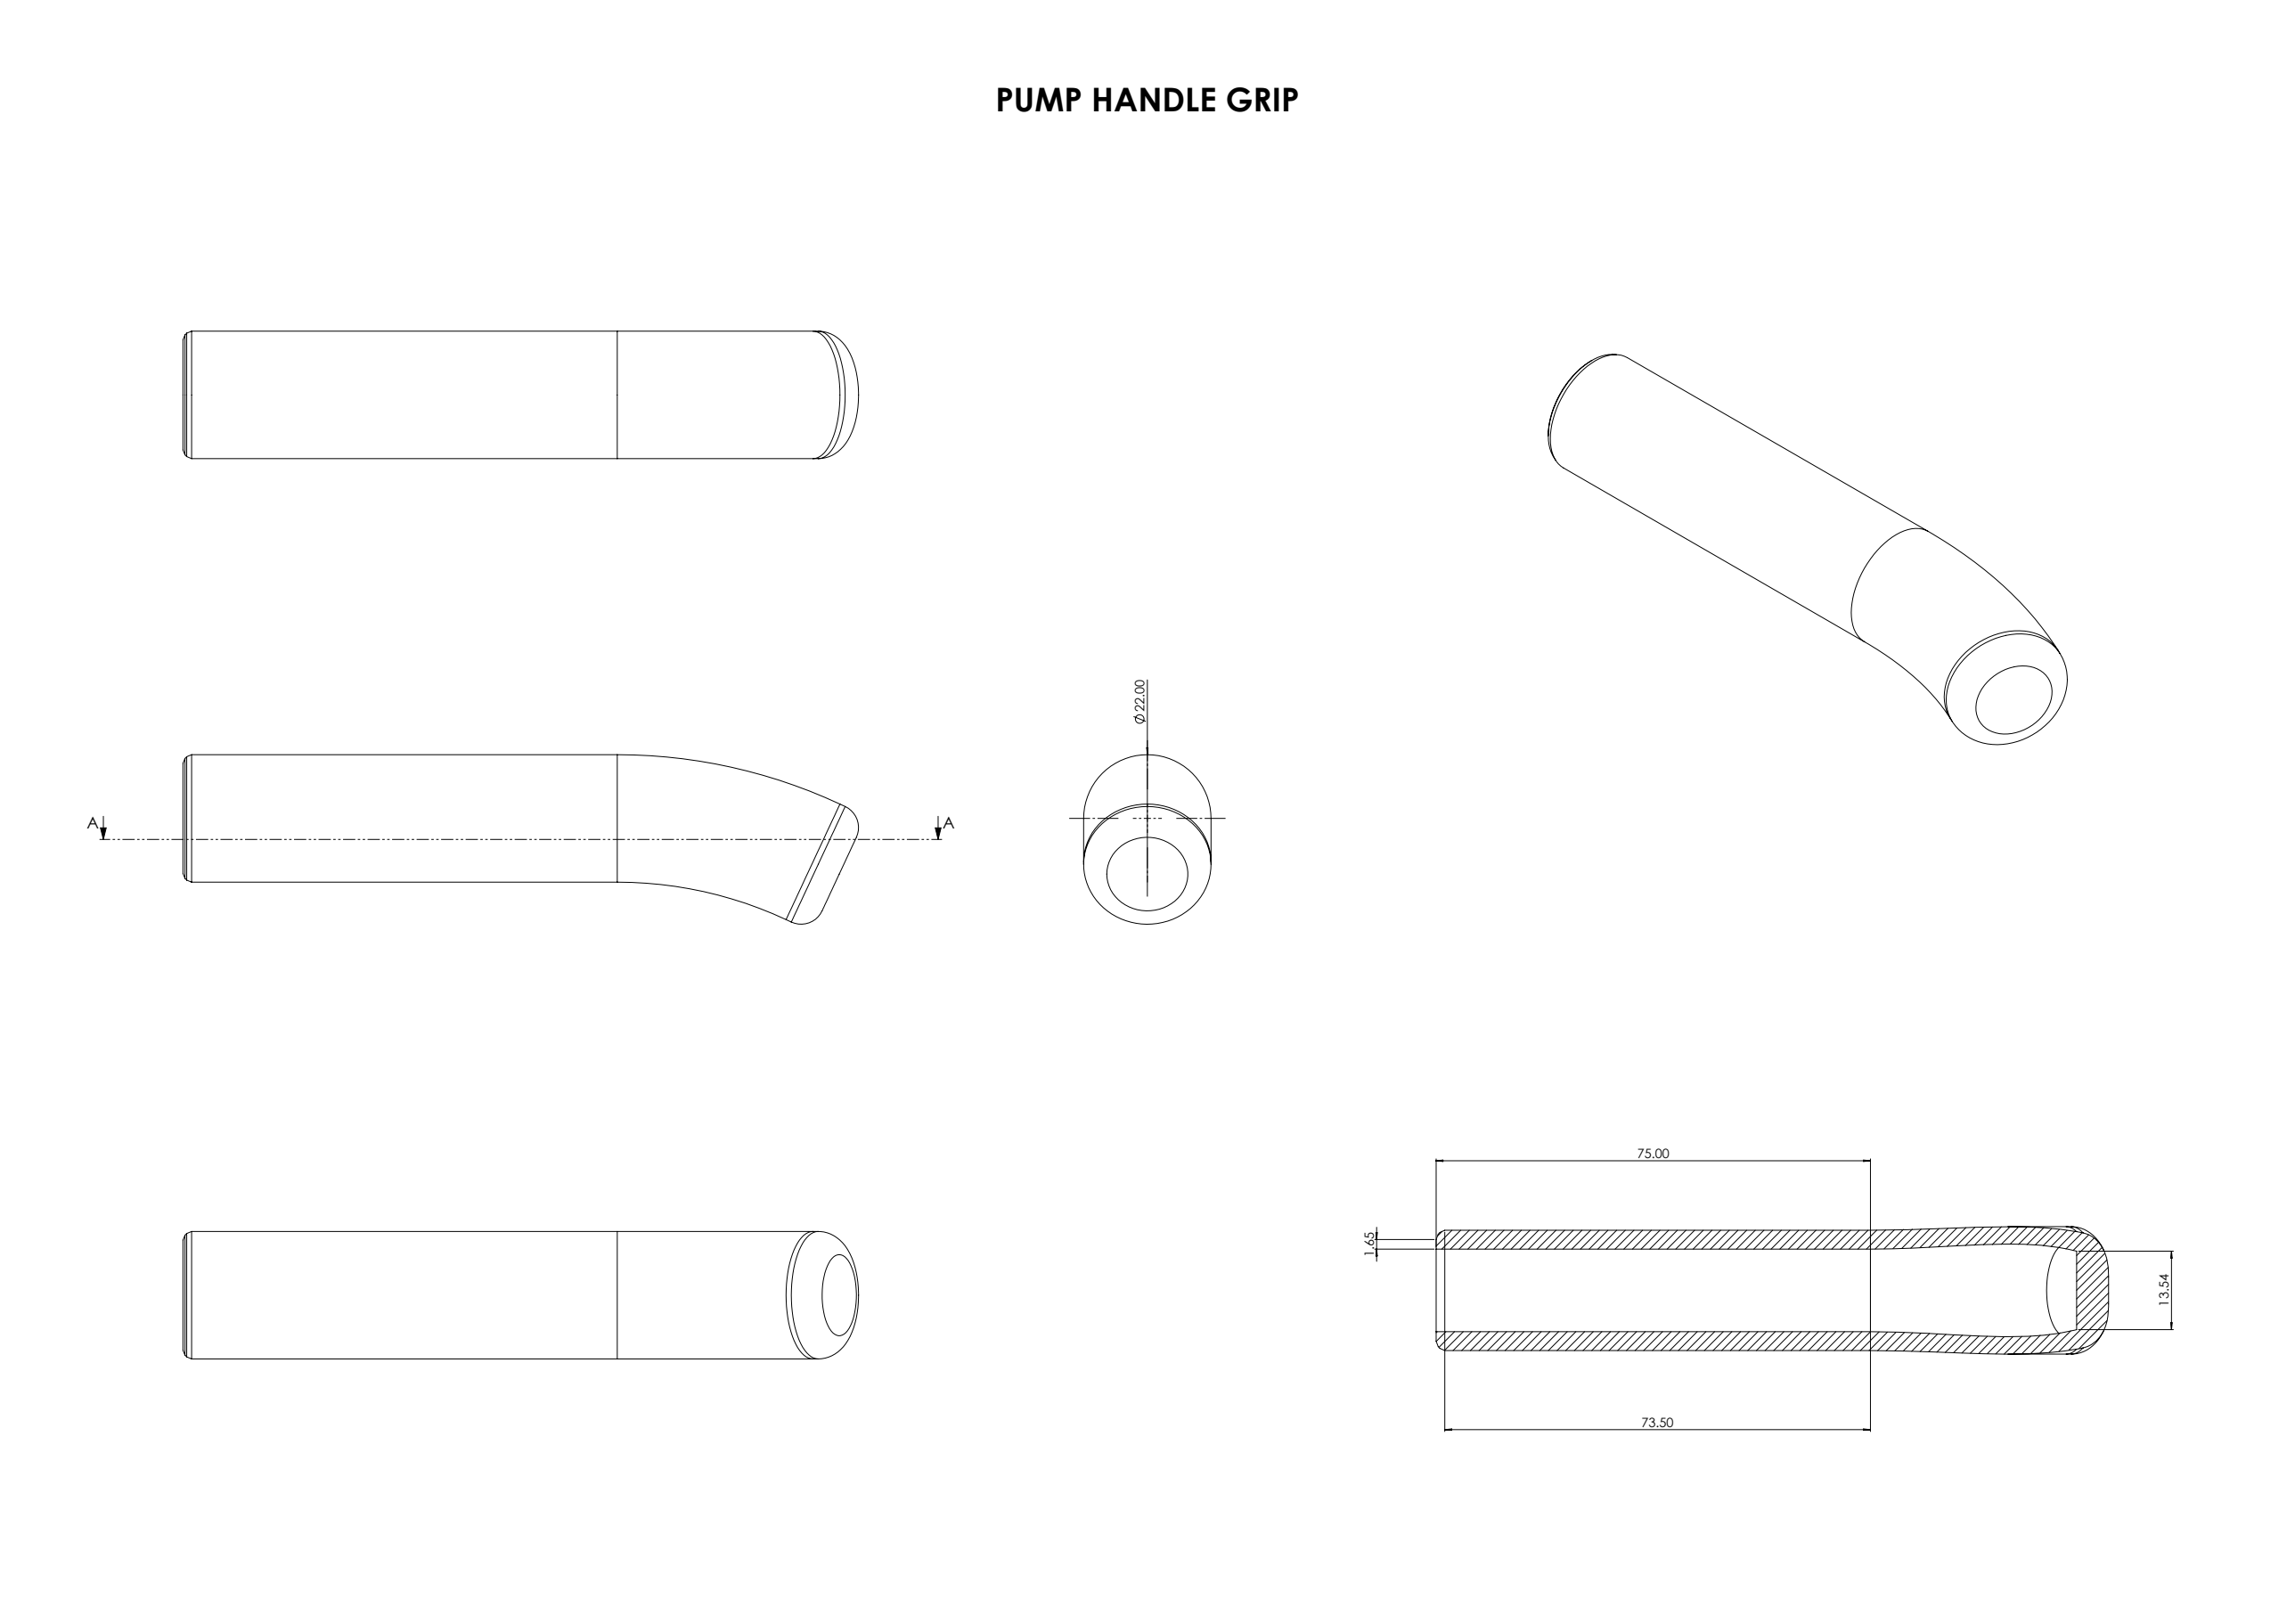
ISO-10303-21;
HEADER;
/* Generated by software containing ST-Developer
 * from STEP Tools, Inc. (www.steptools.com) 
 */

FILE_DESCRIPTION(
/* description */ (''),
/* implementation_level */ '2;1');

FILE_NAME(
/* name */ '15_Pump_Handle_Grip.step',
/* time_stamp */ '2026-10-26T03:55:20-07:00',
/* author */ (''),
/* organization */ (''),
/* preprocessor_version */ 'ST-DEVELOPER v20.2',
/* originating_system */ 'Autodesk Translation Framework v15.15.0.0',
/* authorisation */ '');

FILE_SCHEMA (('AUTOMOTIVE_DESIGN { 1 0 10303 214 3 1 1 }'));
ENDSEC;

DATA;
#10=MECHANICAL_DESIGN_GEOMETRIC_PRESENTATION_REPRESENTATION('',(#190),#45236);
#150=SHAPE_REPRESENTATION_RELATIONSHIP('SRR','None',#45329,#170);
#170=ADVANCED_BREP_SHAPE_REPRESENTATION('',(#210),#45231);
#190=STYLED_ITEM('',(#45491),#210);
#210=MANIFOLD_SOLID_BREP('Body1',#16532);
#228=TOROIDAL_SURFACE('',#17970,7.,4.);
#229=TOROIDAL_SURFACE('',#17981,79.9999999999995,8.);
#230=TOROIDAL_SURFACE('',#17985,79.9999999999995,11.);
#1050=FACE_BOUND('',#3806,.T.);
#1526=PLANE('',#17968);
#1527=PLANE('',#17978);
#1528=PLANE('',#17979);
#1798=CYLINDRICAL_SURFACE('',#17964,11.);
#1799=CYLINDRICAL_SURFACE('',#17975,11.);
#1800=CYLINDRICAL_SURFACE('',#17984,8.);
#2716=FACE_OUTER_BOUND('',#3801,.T.);
#2717=FACE_OUTER_BOUND('',#3802,.T.);
#2718=FACE_OUTER_BOUND('',#3803,.T.);
#2719=FACE_OUTER_BOUND('',#3804,.T.);
#2720=FACE_OUTER_BOUND('',#3805,.T.);
#2721=FACE_OUTER_BOUND('',#3807,.T.);
#2722=FACE_OUTER_BOUND('',#3808,.T.);
#2723=FACE_OUTER_BOUND('',#3809,.T.);
#2724=FACE_OUTER_BOUND('',#3810,.T.);
#2725=FACE_OUTER_BOUND('',#3811,.T.);
#2726=FACE_OUTER_BOUND('',#3812,.T.);
#2727=FACE_OUTER_BOUND('',#3813,.T.);
#3801=EDGE_LOOP('',(#15200,#15201,#15202,#15203));
#3802=EDGE_LOOP('',(#15204,#15205,#15206,#15207));
#3803=EDGE_LOOP('',(#15208,#15209,#15210,#15211));
#3804=EDGE_LOOP('',(#15212,#15213,#15214,#15215));
#3805=EDGE_LOOP('',(#15216));
#3806=EDGE_LOOP('',(#15217));
#3807=EDGE_LOOP('',(#15218,#15219,#15220,#15221,#15222));
#3808=EDGE_LOOP('',(#15223,#15224,#15225,#15226,#15227,#15228));
#3809=EDGE_LOOP('',(#15229));
#3810=EDGE_LOOP('',(#15230));
#3811=EDGE_LOOP('',(#15231,#15232,#15233,#15234));
#3812=EDGE_LOOP('',(#15235,#15236,#15237,#15238));
#3813=EDGE_LOOP('',(#15239,#15240,#15241,#15242,#15243));
#5119=LINE('',#44857,#6430);
#5120=LINE('',#44861,#6431);
#5121=LINE('',#44866,#6432);
#5122=LINE('',#44869,#6433);
#5123=LINE('',#44884,#6434);
#5124=LINE('',#44897,#6435);
#6430=VECTOR('',#21762,10.8232233047034);
#6431=VECTOR('',#21767,10.5);
#6432=VECTOR('',#21774,11.);
#6433=VECTOR('',#21777,9.92677669529664);
#6434=VECTOR('',#21796,11.);
#6435=VECTOR('',#21815,8.);
#6906=CIRCLE('',#17960,10.6464466094067);
#6907=CIRCLE('',#17961,11.);
#6908=CIRCLE('',#17963,10.3535533905933);
#6909=CIRCLE('',#17965,11.);
#6910=CIRCLE('',#17967,9.5);
#6911=CIRCLE('',#17969,8.);
#6912=CIRCLE('',#17971,7.);
#6913=CIRCLE('',#17972,4.);
#6914=CIRCLE('',#17973,11.);
#6915=CIRCLE('',#17974,11.);
#6916=CIRCLE('',#17976,11.);
#6917=CIRCLE('',#17977,11.);
#6918=CIRCLE('',#17980,8.);
#6919=CIRCLE('',#17982,8.);
#6920=CIRCLE('',#17983,71.9999999999995);
#6921=CIRCLE('',#17986,68.9999999999995);
#8382=VERTEX_POINT('',#44854);
#8383=VERTEX_POINT('',#44856);
#8384=VERTEX_POINT('',#44860);
#8385=VERTEX_POINT('',#44864);
#8386=VERTEX_POINT('',#44868);
#8387=VERTEX_POINT('',#44872);
#8388=VERTEX_POINT('',#44875);
#8389=VERTEX_POINT('',#44877);
#8390=VERTEX_POINT('',#44879);
#8391=VERTEX_POINT('',#44883);
#8392=VERTEX_POINT('',#44885);
#8393=VERTEX_POINT('',#44890);
#8394=VERTEX_POINT('',#44893);
#10663=EDGE_CURVE('',#8382,#8382,#6906,.T.);
#10664=EDGE_CURVE('',#8382,#8383,#5119,.T.);
#10665=EDGE_CURVE('',#8383,#8383,#6907,.T.);
#10666=EDGE_CURVE('',#8382,#8384,#5120,.T.);
#10667=EDGE_CURVE('',#8384,#8384,#6908,.T.);
#10668=EDGE_CURVE('',#8385,#8385,#6909,.T.);
#10669=EDGE_CURVE('',#8385,#8383,#5121,.T.);
#10670=EDGE_CURVE('',#8384,#8386,#5122,.T.);
#10671=EDGE_CURVE('',#8386,#8386,#6910,.T.);
#10672=EDGE_CURVE('',#8387,#8387,#6911,.T.);
#10673=EDGE_CURVE('',#8388,#8388,#6912,.T.);
#10674=EDGE_CURVE('',#8388,#8389,#6913,.T.);
#10675=EDGE_CURVE('',#8389,#8390,#6914,.T.);
#10676=EDGE_CURVE('',#8390,#8389,#6915,.T.);
#10677=EDGE_CURVE('',#8390,#8391,#5123,.T.);
#10678=EDGE_CURVE('',#8391,#8392,#6916,.T.);
#10679=EDGE_CURVE('',#8392,#8391,#6917,.T.);
#10680=EDGE_CURVE('',#8393,#8393,#6918,.T.);
#10681=EDGE_CURVE('',#8394,#8394,#6919,.T.);
#10682=EDGE_CURVE('',#8394,#8393,#6920,.T.);
#10683=EDGE_CURVE('',#8387,#8394,#5124,.T.);
#10684=EDGE_CURVE('',#8392,#8385,#6921,.T.);
#15200=ORIENTED_EDGE('',*,*,#10663,.T.);
#15201=ORIENTED_EDGE('',*,*,#10664,.T.);
#15202=ORIENTED_EDGE('',*,*,#10665,.T.);
#15203=ORIENTED_EDGE('',*,*,#10664,.F.);
#15204=ORIENTED_EDGE('',*,*,#10663,.F.);
#15205=ORIENTED_EDGE('',*,*,#10666,.T.);
#15206=ORIENTED_EDGE('',*,*,#10667,.F.);
#15207=ORIENTED_EDGE('',*,*,#10666,.F.);
#15208=ORIENTED_EDGE('',*,*,#10668,.F.);
#15209=ORIENTED_EDGE('',*,*,#10669,.T.);
#15210=ORIENTED_EDGE('',*,*,#10665,.F.);
#15211=ORIENTED_EDGE('',*,*,#10669,.F.);
#15212=ORIENTED_EDGE('',*,*,#10667,.T.);
#15213=ORIENTED_EDGE('',*,*,#10670,.T.);
#15214=ORIENTED_EDGE('',*,*,#10671,.T.);
#15215=ORIENTED_EDGE('',*,*,#10670,.F.);
#15216=ORIENTED_EDGE('',*,*,#10671,.F.);
#15217=ORIENTED_EDGE('',*,*,#10672,.T.);
#15218=ORIENTED_EDGE('',*,*,#10673,.T.);
#15219=ORIENTED_EDGE('',*,*,#10674,.T.);
#15220=ORIENTED_EDGE('',*,*,#10675,.T.);
#15221=ORIENTED_EDGE('',*,*,#10676,.T.);
#15222=ORIENTED_EDGE('',*,*,#10674,.F.);
#15223=ORIENTED_EDGE('',*,*,#10676,.F.);
#15224=ORIENTED_EDGE('',*,*,#10677,.T.);
#15225=ORIENTED_EDGE('',*,*,#10678,.T.);
#15226=ORIENTED_EDGE('',*,*,#10679,.T.);
#15227=ORIENTED_EDGE('',*,*,#10677,.F.);
#15228=ORIENTED_EDGE('',*,*,#10675,.F.);
#15229=ORIENTED_EDGE('',*,*,#10673,.F.);
#15230=ORIENTED_EDGE('',*,*,#10680,.T.);
#15231=ORIENTED_EDGE('',*,*,#10681,.F.);
#15232=ORIENTED_EDGE('',*,*,#10682,.T.);
#15233=ORIENTED_EDGE('',*,*,#10680,.F.);
#15234=ORIENTED_EDGE('',*,*,#10682,.F.);
#15235=ORIENTED_EDGE('',*,*,#10672,.F.);
#15236=ORIENTED_EDGE('',*,*,#10683,.T.);
#15237=ORIENTED_EDGE('',*,*,#10681,.T.);
#15238=ORIENTED_EDGE('',*,*,#10683,.F.);
#15239=ORIENTED_EDGE('',*,*,#10678,.F.);
#15240=ORIENTED_EDGE('',*,*,#10679,.F.);
#15241=ORIENTED_EDGE('',*,*,#10684,.T.);
#15242=ORIENTED_EDGE('',*,*,#10668,.T.);
#15243=ORIENTED_EDGE('',*,*,#10684,.F.);
#15527=CONICAL_SURFACE('',#17959,10.8232233047034,0.392699081698727);
#15528=CONICAL_SURFACE('',#17962,10.5,0.785398163397451);
#15529=CONICAL_SURFACE('',#17966,9.92677669529664,1.17809724509617);
#16444=ADVANCED_FACE('',(#2716),#15527,.T.);
#16445=ADVANCED_FACE('',(#2717),#15528,.T.);
#16446=ADVANCED_FACE('',(#2718),#1798,.T.);
#16447=ADVANCED_FACE('',(#2719),#15529,.T.);
#16448=ADVANCED_FACE('',(#2720,#1050),#1526,.F.);
#16449=ADVANCED_FACE('',(#2721),#228,.T.);
#16450=ADVANCED_FACE('',(#2722),#1799,.T.);
#16451=ADVANCED_FACE('',(#2723),#1527,.F.);
#16452=ADVANCED_FACE('',(#2724),#1528,.T.);
#16453=ADVANCED_FACE('',(#2725),#229,.F.);
#16454=ADVANCED_FACE('',(#2726),#1800,.F.);
#16455=ADVANCED_FACE('',(#2727),#230,.T.);
#16532=CLOSED_SHELL('',(#16444,#16445,#16446,#16447,#16448,#16449,#16450,
#16451,#16452,#16453,#16454,#16455));
#17958=AXIS2_PLACEMENT_3D('',#44852,#21756,#21757);
#17959=AXIS2_PLACEMENT_3D('',#44853,#21758,#21759);
#17960=AXIS2_PLACEMENT_3D('',#44855,#21760,#21761);
#17961=AXIS2_PLACEMENT_3D('',#44858,#21763,#21764);
#17962=AXIS2_PLACEMENT_3D('',#44859,#21765,#21766);
#17963=AXIS2_PLACEMENT_3D('',#44862,#21768,#21769);
#17964=AXIS2_PLACEMENT_3D('',#44863,#21770,#21771);
#17965=AXIS2_PLACEMENT_3D('',#44865,#21772,#21773);
#17966=AXIS2_PLACEMENT_3D('',#44867,#21775,#21776);
#17967=AXIS2_PLACEMENT_3D('',#44870,#21778,#21779);
#17968=AXIS2_PLACEMENT_3D('',#44871,#21780,#21781);
#17969=AXIS2_PLACEMENT_3D('',#44873,#21782,#21783);
#17970=AXIS2_PLACEMENT_3D('',#44874,#21784,#21785);
#17971=AXIS2_PLACEMENT_3D('',#44876,#21786,#21787);
#17972=AXIS2_PLACEMENT_3D('',#44878,#21788,#21789);
#17973=AXIS2_PLACEMENT_3D('',#44880,#21790,#21791);
#17974=AXIS2_PLACEMENT_3D('',#44881,#21792,#21793);
#17975=AXIS2_PLACEMENT_3D('',#44882,#21794,#21795);
#17976=AXIS2_PLACEMENT_3D('',#44886,#21797,#21798);
#17977=AXIS2_PLACEMENT_3D('',#44887,#21799,#21800);
#17978=AXIS2_PLACEMENT_3D('',#44888,#21801,#21802);
#17979=AXIS2_PLACEMENT_3D('',#44889,#21803,#21804);
#17980=AXIS2_PLACEMENT_3D('',#44891,#21805,#21806);
#17981=AXIS2_PLACEMENT_3D('',#44892,#21807,#21808);
#17982=AXIS2_PLACEMENT_3D('',#44894,#21809,#21810);
#17983=AXIS2_PLACEMENT_3D('',#44895,#21811,#21812);
#17984=AXIS2_PLACEMENT_3D('',#44896,#21813,#21814);
#17985=AXIS2_PLACEMENT_3D('',#44898,#21816,#21817);
#17986=AXIS2_PLACEMENT_3D('',#44899,#21818,#21819);
#21756=DIRECTION('axis',(0.,0.,1.));
#21757=DIRECTION('refdir',(1.,0.,0.));
#21758=DIRECTION('center_axis',(1.,7.63756368739912E-16,0.));
#21759=DIRECTION('ref_axis',(0.,3.0116113276618E-17,-1.));
#21760=DIRECTION('center_axis',(1.,0.,0.));
#21761=DIRECTION('ref_axis',(0.,6.12323399573677E-17,-1.));
#21762=DIRECTION('',(0.923879532511286,7.40959143359019E-16,0.382683432365092));
#21763=DIRECTION('center_axis',(-1.,0.,0.));
#21764=DIRECTION('ref_axis',(0.,0.,-1.));
#21765=DIRECTION('center_axis',(1.,0.,0.));
#21766=DIRECTION('ref_axis',(0.,0.,-1.));
#21767=DIRECTION('',(-0.707106781186546,8.65956056235495E-17,-0.707106781186549));
#21768=DIRECTION('center_axis',(-1.,0.,0.));
#21769=DIRECTION('ref_axis',(0.,6.12323399573677E-17,-1.));
#21770=DIRECTION('center_axis',(1.,0.,0.));
#21771=DIRECTION('ref_axis',(0.,0.,-1.));
#21772=DIRECTION('center_axis',(1.,0.,0.));
#21773=DIRECTION('ref_axis',(0.,0.,-1.));
#21774=DIRECTION('',(-1.,0.,0.));
#21775=DIRECTION('center_axis',(1.,-1.79314445242836E-15,0.));
#21776=DIRECTION('ref_axis',(0.,3.1932434889965E-17,-1.));
#21777=DIRECTION('',(-0.382683432365088,8.28851008028559E-16,-0.923879532511287));
#21778=DIRECTION('center_axis',(1.,0.,0.));
#21779=DIRECTION('ref_axis',(0.,0.,-1.));
#21780=DIRECTION('center_axis',(1.,0.,0.));
#21781=DIRECTION('ref_axis',(0.,0.,-1.));
#21782=DIRECTION('center_axis',(1.,0.,0.));
#21783=DIRECTION('ref_axis',(0.,0.,-1.));
#21784=DIRECTION('center_axis',(0.906307787036649,-6.16297582203915E-33,
0.422618261740701));
#21785=DIRECTION('ref_axis',(0.422618261740702,0.,-0.906307787036649));
#21786=DIRECTION('center_axis',(-0.906307787036649,6.16297582203915E-33,
-0.422618261740701));
#21787=DIRECTION('ref_axis',(2.06315799195206E-17,1.,-4.42445659184577E-17));
#21788=DIRECTION('center_axis',(5.17558101501968E-17,-1.,-1.10990693043675E-16));
#21789=DIRECTION('ref_axis',(-0.422618261740701,-1.22464679914735E-16,0.906307787036649));
#21790=DIRECTION('center_axis',(0.906307787036649,-6.16297582203915E-33,
0.422618261740701));
#21791=DIRECTION('ref_axis',(-1.00929365875014E-16,1.,-1.00929365875014E-16));
#21792=DIRECTION('center_axis',(0.906307787036649,-6.16297582203915E-33,
0.422618261740701));
#21793=DIRECTION('ref_axis',(-1.00929365875014E-16,1.,-1.00929365875014E-16));
#21794=DIRECTION('center_axis',(0.90630778703665,0.,0.422618261740699));
#21795=DIRECTION('ref_axis',(-5.17558101501966E-17,1.,1.10990693043675E-16));
#21796=DIRECTION('',(-0.90630778703665,0.,-0.422618261740699));
#21797=DIRECTION('center_axis',(0.906307787036649,0.,0.422618261740702));
#21798=DIRECTION('ref_axis',(0.422618261740702,0.,-0.906307787036649));
#21799=DIRECTION('center_axis',(0.906307787036649,0.,0.422618261740702));
#21800=DIRECTION('ref_axis',(0.422618261740702,0.,-0.906307787036649));
#21801=DIRECTION('center_axis',(-0.906307787036649,6.16297582203915E-33,
-0.422618261740701));
#21802=DIRECTION('ref_axis',(-5.17558101501968E-17,1.,1.10990693043675E-16));
#21803=DIRECTION('center_axis',(-0.906307787036649,6.16297582203915E-33,
-0.422618261740701));
#21804=DIRECTION('ref_axis',(-5.17558101501968E-17,1.,1.10990693043675E-16));
#21805=DIRECTION('center_axis',(-0.906307787036649,0.,-0.422618261740702));
#21806=DIRECTION('ref_axis',(0.422618261740701,0.,-0.906307787036649));
#21807=DIRECTION('center_axis',(0.,-1.,0.));
#21808=DIRECTION('ref_axis',(0.,0.,-1.));
#21809=DIRECTION('center_axis',(1.,0.,0.));
#21810=DIRECTION('ref_axis',(0.,0.,-1.));
#21811=DIRECTION('center_axis',(0.,-1.,0.));
#21812=DIRECTION('ref_axis',(0.,0.,-1.));
#21813=DIRECTION('center_axis',(1.,0.,0.));
#21814=DIRECTION('ref_axis',(0.,0.,-1.));
#21815=DIRECTION('',(1.,0.,0.));
#21816=DIRECTION('center_axis',(0.,-1.,0.));
#21817=DIRECTION('ref_axis',(0.,0.,-1.));
#21818=DIRECTION('center_axis',(0.,1.,0.));
#21819=DIRECTION('ref_axis',(0.,0.,-1.));
#44852=CARTESIAN_POINT('',(0.,0.,0.));
#44853=CARTESIAN_POINT('Origin',(76.0732233047034,-3.25953419062578E-16,
0.));
#44854=CARTESIAN_POINT('',(75.6464466094067,-2.60762735250063E-15,10.6464466094067));
#44855=CARTESIAN_POINT('Origin',(75.6464466094067,-6.51906838125157E-16,
0.));
#44856=CARTESIAN_POINT('',(76.5,1.34711147906209E-15,11.));
#44857=CARTESIAN_POINT('',(76.0732233047034,6.73555739531044E-16,10.8232233047034));
#44858=CARTESIAN_POINT('Origin',(76.5,0.,0.));
#44859=CARTESIAN_POINT('Origin',(75.5,0.,0.));
#44860=CARTESIAN_POINT('',(75.3535533905933,0.,10.3535533905933));
#44861=CARTESIAN_POINT('',(75.5,-1.28587913910472E-15,10.5));
#44862=CARTESIAN_POINT('Origin',(75.3535533905933,-6.33972300979564E-16,
0.));
#44863=CARTESIAN_POINT('Origin',(75.,0.,0.));
#44864=CARTESIAN_POINT('',(150.,-1.34711147906209E-15,11.));
#44865=CARTESIAN_POINT('Origin',(150.,0.,0.));
#44866=CARTESIAN_POINT('',(75.,-1.34711147906209E-15,11.));
#44867=CARTESIAN_POINT('Origin',(75.1767766952966,-3.16986150489782E-16,
0.));
#44868=CARTESIAN_POINT('',(75.,-1.16341445918999E-15,9.5));
#44869=CARTESIAN_POINT('',(75.1767766952966,-1.84965183155412E-15,9.92677669529664));
#44870=CARTESIAN_POINT('Origin',(75.,0.,0.));
#44871=CARTESIAN_POINT('Origin',(75.,0.,0.));
#44872=CARTESIAN_POINT('',(75.,-9.79717439317883E-16,8.));
#44873=CARTESIAN_POINT('Origin',(75.,0.,0.));
#44874=CARTESIAN_POINT('Origin',(184.715768726293,8.84447404295016E-31,
7.91799529880872));
#44875=CARTESIAN_POINT('',(185.382672042254,-8.57252759403147E-16,15.9526228550281));
#44876=CARTESIAN_POINT('Origin',(188.340999874439,8.5979550100686E-31,9.60846834577153));
#44877=CARTESIAN_POINT('',(180.066967847145,-1.34711147906209E-15,17.8873809562119));
#44878=CARTESIAN_POINT('Origin',(181.757440894108,-8.57252759403146E-16,
14.2621498080653));
#44879=CARTESIAN_POINT('',(184.715768726293,-11.,7.91799529880872));
#44880=CARTESIAN_POINT('Origin',(184.715768726293,8.84447404295016E-31,
7.91799529880872));
#44881=CARTESIAN_POINT('Origin',(184.715768726293,8.84447404295016E-31,
7.91799529880872));
#44882=CARTESIAN_POINT('Origin',(183.809460939256,8.84447404295016E-31,
7.49537703706802));
#44883=CARTESIAN_POINT('',(183.809460939256,-11.,7.49537703706799));
#44884=CARTESIAN_POINT('',(183.809460939256,-11.,7.49537703706802));
#44885=CARTESIAN_POINT('',(179.160660060108,1.34711147906209E-15,17.4647626944711));
#44886=CARTESIAN_POINT('Origin',(183.809460939256,0.,7.49537703706801));
#44887=CARTESIAN_POINT('Origin',(183.809460939256,0.,7.49537703706801));
#44888=CARTESIAN_POINT('Origin',(188.340999874439,-1.08770485875751E-30,
9.60846834577153));
#44889=CARTESIAN_POINT('Origin',(183.809460939256,-1.08770485875751E-30,
7.49537703706802));
#44890=CARTESIAN_POINT('',(180.42851484533,-9.79717439317883E-16,14.7458393333612));
#44891=CARTESIAN_POINT('Origin',(183.809460939256,0.,7.49537703706803));
#44892=CARTESIAN_POINT('Origin',(150.,0.,79.9999999999995));
#44893=CARTESIAN_POINT('',(150.,-9.79717439317883E-16,8.));
#44894=CARTESIAN_POINT('Origin',(150.,0.,0.));
#44895=CARTESIAN_POINT('Origin',(150.,9.79717439317883E-16,79.9999999999995));
#44896=CARTESIAN_POINT('Origin',(75.,0.,0.));
#44897=CARTESIAN_POINT('',(75.,-9.79717439317883E-16,8.));
#44898=CARTESIAN_POINT('Origin',(150.,0.,79.9999999999995));
#44899=CARTESIAN_POINT('Origin',(150.,1.34711147906209E-15,79.9999999999995));
#45209=UNCERTAINTY_MEASURE_WITH_UNIT(LENGTH_MEASURE(0.01),#45237,
'DISTANCE_ACCURACY_VALUE',
'Maximum model space distance between geometric entities at asserted c
onnectivities');
#45214=UNCERTAINTY_MEASURE_WITH_UNIT(LENGTH_MEASURE(0.01),#45237,
'DISTANCE_ACCURACY_VALUE',
'Maximum model space distance between geometric entities at asserted c
onnectivities');
#45231=(
GEOMETRIC_REPRESENTATION_CONTEXT(3)
GLOBAL_UNCERTAINTY_ASSIGNED_CONTEXT((#45209))
GLOBAL_UNIT_ASSIGNED_CONTEXT((#45237,#45239,#45240))
REPRESENTATION_CONTEXT('','3D')
);
#45236=(
GEOMETRIC_REPRESENTATION_CONTEXT(3)
GLOBAL_UNCERTAINTY_ASSIGNED_CONTEXT((#45214))
GLOBAL_UNIT_ASSIGNED_CONTEXT((#45237,#45239,#45240))
REPRESENTATION_CONTEXT('','3D')
);
#45237=(
LENGTH_UNIT()
NAMED_UNIT(*)
SI_UNIT(.MILLI.,.METRE.)
);
#45239=(
NAMED_UNIT(*)
PLANE_ANGLE_UNIT()
SI_UNIT($,.RADIAN.)
);
#45240=(
NAMED_UNIT(*)
SI_UNIT($,.STERADIAN.)
SOLID_ANGLE_UNIT()
);
#45257=SHAPE_DEFINITION_REPRESENTATION(#45278,#45329);
#45278=PRODUCT_DEFINITION_SHAPE('',$,#45351);
#45329=SHAPE_REPRESENTATION('',(#17958),#45231);
#45334=PRODUCT_DEFINITION_CONTEXT('part definition',#45399,'design');
#45351=PRODUCT_DEFINITION('2026-10-25-23-38-24-602',
'15_Pump_Handle_Grip',#45372,#45334);
#45372=PRODUCT_DEFINITION_FORMATION('',$,#45417);
#45399=APPLICATION_CONTEXT(
'Core Data for Automotive Mechanical Design Process');
#45400=PRODUCT_CONTEXT('part definition',#45399,'mechanical');
#45417=PRODUCT('2026-10-25-23-38-24-602','15_Pump_Handle_Grip',$,(#45400));
#45485=COLOUR_RGB('Black',0.12,0.14,0.17);
#45486=FILL_AREA_STYLE_COLOUR('',#45485);
#45487=FILL_AREA_STYLE('',(#45486));
#45488=SURFACE_STYLE_FILL_AREA(#45487);
#45489=SURFACE_SIDE_STYLE('',(#45488));
#45490=SURFACE_STYLE_USAGE(.BOTH.,#45489);
#45491=PRESENTATION_STYLE_ASSIGNMENT((#45490));
ENDSEC;
END-ISO-10303-21;
